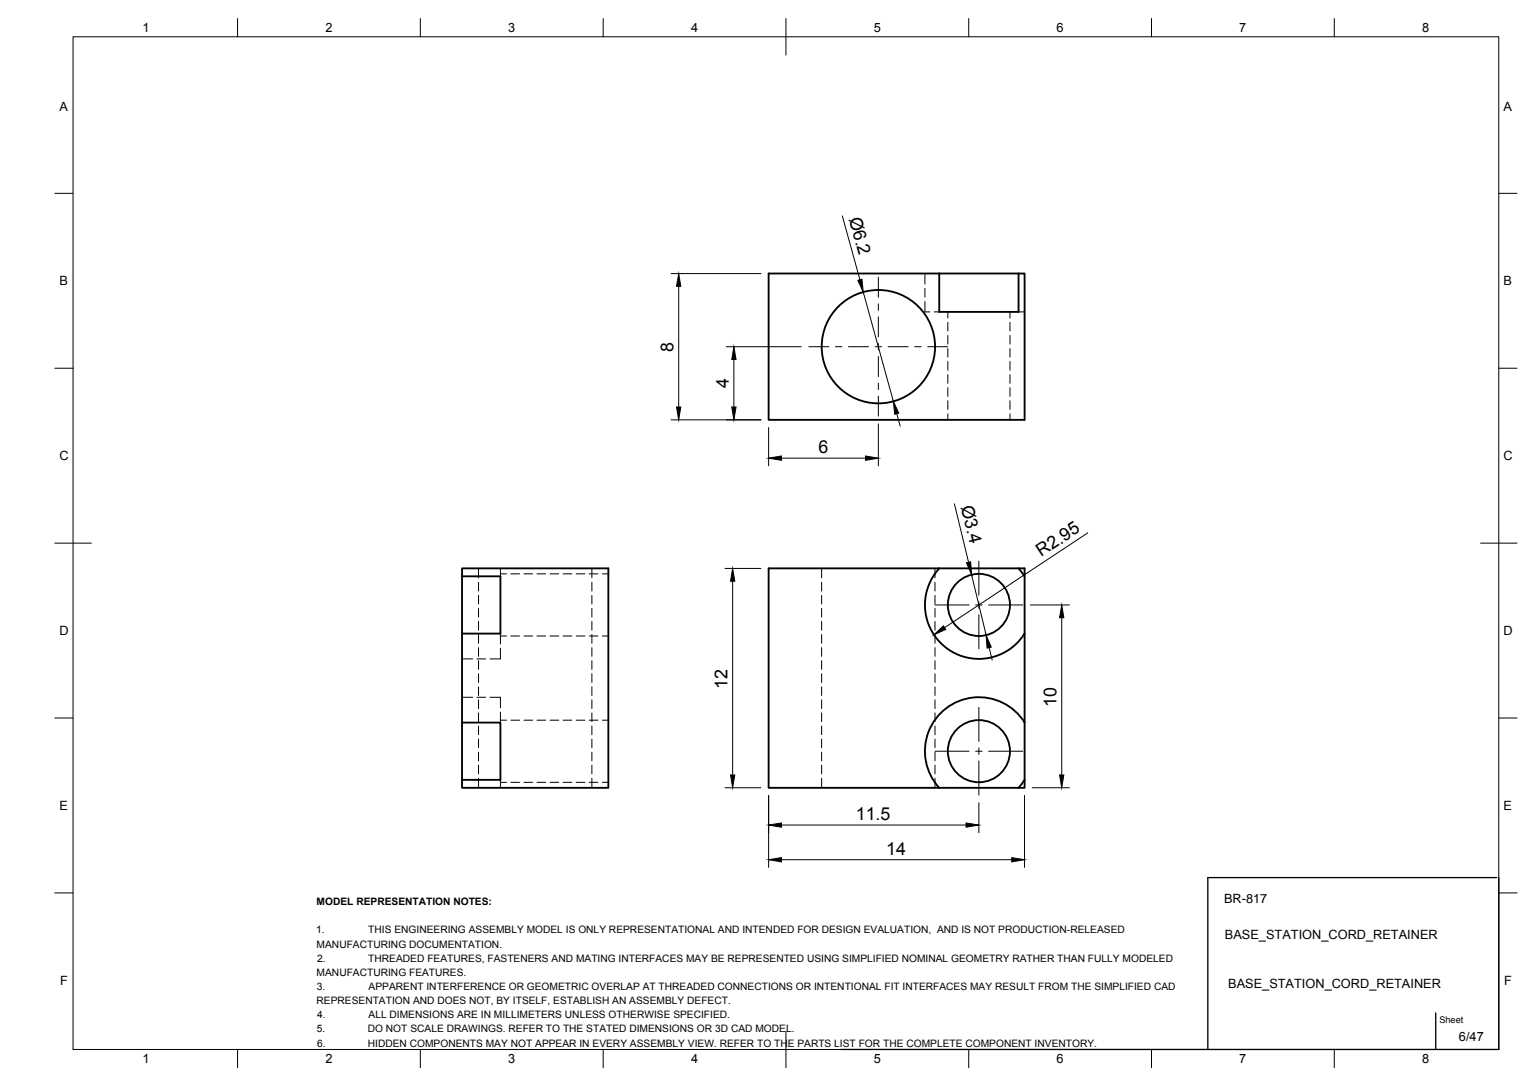
ISO-10303-21;
HEADER;
FILE_DESCRIPTION((''),'2;1');
FILE_NAME('BASE_STATION_CORD_RETAINER.step','2026-10-01T22:07:29-07:00',(''),(''),'','','');
FILE_SCHEMA (('AUTOMOTIVE_DESIGN { 1 0 10303 214 3 1 1 }'));
ENDSEC;
DATA;
#10=MECHANICAL_DESIGN_GEOMETRIC_PRESENTATION_REPRESENTATION('',(#544),#15484);
#474=SHAPE_REPRESENTATION_RELATIONSHIP('SRR','None',#15621,#509) ;
#509=ADVANCED_BREP_SHAPE_REPRESENTATION('',(#586),#15445) ;
#544=STYLED_ITEM('',(#15833),#586) ;
#586=MANIFOLD_SOLID_BREP('BASE_STATION_CORD_RETAINER',#8253) ;
#639=CYLINDRICAL_SURFACE('',#8765,0.295) ;
#640=CYLINDRICAL_SURFACE('',#8771,0.295) ;
#641=CYLINDRICAL_SURFACE('',#8776,0.17) ;
#642=CYLINDRICAL_SURFACE('',#8778,0.295) ;
#643=CYLINDRICAL_SURFACE('',#8781,0.295) ;
#644=CYLINDRICAL_SURFACE('',#8789,0.17) ;
#645=CYLINDRICAL_SURFACE('',#8791,0.31) ;
#831=FACE_BOUND('',#1941,.T.) ;
#832=FACE_BOUND('',#1944,.T.) ;
#833=FACE_BOUND('',#1950,.T.) ;
#834=FACE_BOUND('',#1957,.T.) ;
#835=FACE_BOUND('',#1958,.T.) ;
#836=FACE_BOUND('',#1961,.T.) ;
#911=CIRCLE('',#8766,0.295) ;
#912=CIRCLE('',#8767,0.295) ;
#913=CIRCLE('',#8769,0.295) ;
#914=CIRCLE('',#8770,0.17) ;
#915=CIRCLE('',#8772,0.295) ;
#916=CIRCLE('',#8774,0.31) ;
#917=CIRCLE('',#8777,0.17) ;
#918=CIRCLE('',#8779,0.295) ;
#919=CIRCLE('',#8780,0.295) ;
#920=CIRCLE('',#8782,0.295) ;
#921=CIRCLE('',#8783,0.295) ;
#922=CIRCLE('',#8785,0.17) ;
#923=CIRCLE('',#8790,0.17) ;
#924=CIRCLE('',#8792,0.31) ;
#1418=FACE_OUTER_BOUND('',#1939,.T.) ;
#1419=FACE_OUTER_BOUND('',#1940,.T.) ;
#1420=FACE_OUTER_BOUND('',#1942,.T.) ;
#1421=FACE_OUTER_BOUND('',#1943,.T.) ;
#1422=FACE_OUTER_BOUND('',#1945,.T.) ;
#1423=FACE_OUTER_BOUND('',#1946,.T.) ;
#1424=FACE_OUTER_BOUND('',#1947,.T.) ;
#1425=FACE_OUTER_BOUND('',#1948,.T.) ;
#1426=FACE_OUTER_BOUND('',#1949,.T.) ;
#1427=FACE_OUTER_BOUND('',#1951,.T.) ;
#1428=FACE_OUTER_BOUND('',#1952,.T.) ;
#1429=FACE_OUTER_BOUND('',#1953,.T.) ;
#1430=FACE_OUTER_BOUND('',#1954,.T.) ;
#1431=FACE_OUTER_BOUND('',#1955,.T.) ;
#1432=FACE_OUTER_BOUND('',#1956,.T.) ;
#1433=FACE_OUTER_BOUND('',#1959,.T.) ;
#1434=FACE_OUTER_BOUND('',#1960,.T.) ;
#1939=EDGE_LOOP('',(#5513,#5514,#5515,#5516)) ;
#1940=EDGE_LOOP('',(#5517,#5518,#5519,#5520)) ;
#1941=EDGE_LOOP('',(#5521)) ;
#1942=EDGE_LOOP('',(#5522,#5523,#5524,#5525)) ;
#1943=EDGE_LOOP('',(#5526,#5527,#5528,#5529,#5530,#5531,#5532,#5533)) ;
#1944=EDGE_LOOP('',(#5534)) ;
#1945=EDGE_LOOP('',(#5535,#5536,#5537)) ;
#1946=EDGE_LOOP('',(#5538,#5539,#5540,#5541)) ;
#1947=EDGE_LOOP('',(#5542,#5543,#5544,#5545)) ;
#1948=EDGE_LOOP('',(#5546,#5547,#5548,#5549)) ;
#1949=EDGE_LOOP('',(#5550,#5551,#5552,#5553)) ;
#1950=EDGE_LOOP('',(#5554)) ;
#1951=EDGE_LOOP('',(#5555,#5556,#5557,#5558,#5559,#5560,#5561,#5562,#5563,
#5564,#5565,#5566)) ;
#1952=EDGE_LOOP('',(#5567,#5568,#5569)) ;
#1953=EDGE_LOOP('',(#5570,#5571,#5572,#5573,#5574,#5575)) ;
#1954=EDGE_LOOP('',(#5576,#5577,#5578,#5579)) ;
#1955=EDGE_LOOP('',(#5580,#5581,#5582,#5583)) ;
#1956=EDGE_LOOP('',(#5584,#5585,#5586,#5587)) ;
#1957=EDGE_LOOP('',(#5588)) ;
#1958=EDGE_LOOP('',(#5589)) ;
#1959=EDGE_LOOP('',(#5590,#5591,#5592,#5593)) ;
#1960=EDGE_LOOP('',(#5594,#5595,#5596,#5597,#5598,#5599,#5600,#5601)) ;
#1961=EDGE_LOOP('',(#5602)) ;
#2534=LINE('',#13145,#3008) ;
#2535=LINE('',#13149,#3009) ;
#2536=LINE('',#13153,#3010) ;
#2537=LINE('',#13156,#3011) ;
#2538=LINE('',#13161,#3012) ;
#2539=LINE('',#13164,#3013) ;
#2540=LINE('',#13167,#3014) ;
#2541=LINE('',#13169,#3015) ;
#2542=LINE('',#13171,#3016) ;
#2543=LINE('',#13173,#3017) ;
#2544=LINE('',#13174,#3018) ;
#2545=LINE('',#13178,#3019) ;
#2546=LINE('',#13181,#3020) ;
#2547=LINE('',#13186,#3021) ;
#2548=LINE('',#13190,#3022) ;
#2549=LINE('',#13195,#3023) ;
#2550=LINE('',#13199,#3024) ;
#2551=LINE('',#13202,#3025) ;
#2552=LINE('',#13203,#3026) ;
#2553=LINE('',#13207,#3027) ;
#2554=LINE('',#13209,#3028) ;
#2555=LINE('',#13211,#3029) ;
#2556=LINE('',#13212,#3030) ;
#2557=LINE('',#13214,#3031) ;
#2558=LINE('',#13217,#3032) ;
#2559=LINE('',#13218,#3033) ;
#2560=LINE('',#13221,#3034) ;
#2561=LINE('',#13226,#3035) ;
#2562=LINE('',#13229,#3036) ;
#2563=LINE('',#13230,#3037) ;
#2564=LINE('',#13232,#3038) ;
#3008=VECTOR('',#10187,1.) ;
#3009=VECTOR('',#10190,1.) ;
#3010=VECTOR('',#10195,1.) ;
#3011=VECTOR('',#10198,1.) ;
#3012=VECTOR('',#10203,1.) ;
#3013=VECTOR('',#10206,1.) ;
#3014=VECTOR('',#10209,1.) ;
#3015=VECTOR('',#10210,1.) ;
#3016=VECTOR('',#10211,1.) ;
#3017=VECTOR('',#10212,1.) ;
#3018=VECTOR('',#10213,1.) ;
#3019=VECTOR('',#10218,1.) ;
#3020=VECTOR('',#10221,0.17) ;
#3021=VECTOR('',#10226,1.) ;
#3022=VECTOR('',#10229,1.) ;
#3023=VECTOR('',#10234,1.) ;
#3024=VECTOR('',#10237,1.) ;
#3025=VECTOR('',#10242,1.) ;
#3026=VECTOR('',#10243,1.) ;
#3027=VECTOR('',#10248,1.) ;
#3028=VECTOR('',#10249,1.) ;
#3029=VECTOR('',#10250,1.) ;
#3030=VECTOR('',#10251,1.) ;
#3031=VECTOR('',#10254,1.) ;
#3032=VECTOR('',#10257,1.) ;
#3033=VECTOR('',#10258,1.) ;
#3034=VECTOR('',#10261,0.17) ;
#3035=VECTOR('',#10268,0.31) ;
#3036=VECTOR('',#10271,1.) ;
#3037=VECTOR('',#10272,1.) ;
#3038=VECTOR('',#10275,1.) ;
#3468=VERTEX_POINT('',#13143) ;
#3469=VERTEX_POINT('',#13144) ;
#3470=VERTEX_POINT('',#13146) ;
#3471=VERTEX_POINT('',#13148) ;
#3472=VERTEX_POINT('',#13152) ;
#3473=VERTEX_POINT('',#13154) ;
#3474=VERTEX_POINT('',#13157) ;
#3475=VERTEX_POINT('',#13160) ;
#3476=VERTEX_POINT('',#13162) ;
#3477=VERTEX_POINT('',#13166) ;
#3478=VERTEX_POINT('',#13168) ;
#3479=VERTEX_POINT('',#13170) ;
#3480=VERTEX_POINT('',#13172) ;
#3481=VERTEX_POINT('',#13175) ;
#3482=VERTEX_POINT('',#13180) ;
#3483=VERTEX_POINT('',#13184) ;
#3484=VERTEX_POINT('',#13185) ;
#3485=VERTEX_POINT('',#13187) ;
#3486=VERTEX_POINT('',#13189) ;
#3487=VERTEX_POINT('',#13193) ;
#3488=VERTEX_POINT('',#13194) ;
#3489=VERTEX_POINT('',#13196) ;
#3490=VERTEX_POINT('',#13198) ;
#3491=VERTEX_POINT('',#13204) ;
#3492=VERTEX_POINT('',#13208) ;
#3493=VERTEX_POINT('',#13210) ;
#3494=VERTEX_POINT('',#13216) ;
#3495=VERTEX_POINT('',#13220) ;
#3496=VERTEX_POINT('',#13224) ;
#3497=VERTEX_POINT('',#13228) ;
#4261=EDGE_CURVE('',#3468,#3469,#2534,.T.) ;
#4262=EDGE_CURVE('',#3468,#3470,#911,.T.) ;
#4263=EDGE_CURVE('',#3471,#3470,#2535,.T.) ;
#4264=EDGE_CURVE('',#3469,#3471,#912,.T.) ;
#4265=EDGE_CURVE('',#3472,#3468,#2536,.T.) ;
#4266=EDGE_CURVE('',#3473,#3472,#913,.T.) ;
#4267=EDGE_CURVE('',#3470,#3473,#2537,.T.) ;
#4268=EDGE_CURVE('',#3474,#3474,#914,.T.) ;
#4269=EDGE_CURVE('',#3475,#3472,#2538,.T.) ;
#4270=EDGE_CURVE('',#3476,#3475,#915,.T.) ;
#4271=EDGE_CURVE('',#3473,#3476,#2539,.T.) ;
#4272=EDGE_CURVE('',#3477,#3469,#2540,.T.) ;
#4273=EDGE_CURVE('',#3478,#3477,#2541,.T.) ;
#4274=EDGE_CURVE('',#3479,#3478,#2542,.T.) ;
#4275=EDGE_CURVE('',#3479,#3480,#2543,.T.) ;
#4276=EDGE_CURVE('',#3475,#3480,#2544,.T.) ;
#4277=EDGE_CURVE('',#3481,#3481,#916,.T.) ;
#4278=EDGE_CURVE('',#3471,#3477,#2545,.T.) ;
#4279=EDGE_CURVE('',#3474,#3482,#2546,.T.) ;
#4280=EDGE_CURVE('',#3482,#3482,#917,.T.) ;
#4281=EDGE_CURVE('',#3483,#3484,#2547,.T.) ;
#4282=EDGE_CURVE('',#3485,#3483,#918,.T.) ;
#4283=EDGE_CURVE('',#3486,#3485,#2548,.T.) ;
#4284=EDGE_CURVE('',#3486,#3484,#919,.T.) ;
#4285=EDGE_CURVE('',#3487,#3488,#2549,.T.) ;
#4286=EDGE_CURVE('',#3487,#3489,#920,.T.) ;
#4287=EDGE_CURVE('',#3490,#3489,#2550,.T.) ;
#4288=EDGE_CURVE('',#3488,#3490,#921,.T.) ;
#4289=EDGE_CURVE('',#3484,#3487,#2551,.T.) ;
#4290=EDGE_CURVE('',#3489,#3486,#2552,.T.) ;
#4291=EDGE_CURVE('',#3491,#3491,#922,.T.) ;
#4292=EDGE_CURVE('',#3490,#3476,#2553,.T.) ;
#4293=EDGE_CURVE('',#3492,#3485,#2554,.T.) ;
#4294=EDGE_CURVE('',#3493,#3492,#2555,.T.) ;
#4295=EDGE_CURVE('',#3478,#3493,#2556,.T.) ;
#4296=EDGE_CURVE('',#3483,#3492,#2557,.T.) ;
#4297=EDGE_CURVE('',#3480,#3494,#2558,.T.) ;
#4298=EDGE_CURVE('',#3494,#3488,#2559,.T.) ;
#4299=EDGE_CURVE('',#3491,#3495,#2560,.T.) ;
#4300=EDGE_CURVE('',#3495,#3495,#923,.T.) ;
#4301=EDGE_CURVE('',#3496,#3496,#924,.T.) ;
#4302=EDGE_CURVE('',#3496,#3481,#2561,.T.) ;
#4303=EDGE_CURVE('',#3493,#3497,#2562,.T.) ;
#4304=EDGE_CURVE('',#3497,#3479,#2563,.T.) ;
#4305=EDGE_CURVE('',#3497,#3494,#2564,.T.) ;
#5513=ORIENTED_EDGE('',*,*,#4261,.F.) ;
#5514=ORIENTED_EDGE('',*,*,#4262,.T.) ;
#5515=ORIENTED_EDGE('',*,*,#4263,.F.) ;
#5516=ORIENTED_EDGE('',*,*,#4264,.F.) ;
#5517=ORIENTED_EDGE('',*,*,#4265,.F.) ;
#5518=ORIENTED_EDGE('',*,*,#4266,.F.) ;
#5519=ORIENTED_EDGE('',*,*,#4267,.F.) ;
#5520=ORIENTED_EDGE('',*,*,#4262,.F.) ;
#5521=ORIENTED_EDGE('',*,*,#4268,.F.) ;
#5522=ORIENTED_EDGE('',*,*,#4269,.F.) ;
#5523=ORIENTED_EDGE('',*,*,#4270,.F.) ;
#5524=ORIENTED_EDGE('',*,*,#4271,.F.) ;
#5525=ORIENTED_EDGE('',*,*,#4266,.T.) ;
#5526=ORIENTED_EDGE('',*,*,#4269,.T.) ;
#5527=ORIENTED_EDGE('',*,*,#4265,.T.) ;
#5528=ORIENTED_EDGE('',*,*,#4261,.T.) ;
#5529=ORIENTED_EDGE('',*,*,#4272,.F.) ;
#5530=ORIENTED_EDGE('',*,*,#4273,.F.) ;
#5531=ORIENTED_EDGE('',*,*,#4274,.F.) ;
#5532=ORIENTED_EDGE('',*,*,#4275,.T.) ;
#5533=ORIENTED_EDGE('',*,*,#4276,.F.) ;
#5534=ORIENTED_EDGE('',*,*,#4277,.T.) ;
#5535=ORIENTED_EDGE('',*,*,#4264,.T.) ;
#5536=ORIENTED_EDGE('',*,*,#4278,.T.) ;
#5537=ORIENTED_EDGE('',*,*,#4272,.T.) ;
#5538=ORIENTED_EDGE('',*,*,#4268,.T.) ;
#5539=ORIENTED_EDGE('',*,*,#4279,.T.) ;
#5540=ORIENTED_EDGE('',*,*,#4280,.F.) ;
#5541=ORIENTED_EDGE('',*,*,#4279,.F.) ;
#5542=ORIENTED_EDGE('',*,*,#4281,.F.) ;
#5543=ORIENTED_EDGE('',*,*,#4282,.F.) ;
#5544=ORIENTED_EDGE('',*,*,#4283,.F.) ;
#5545=ORIENTED_EDGE('',*,*,#4284,.T.) ;
#5546=ORIENTED_EDGE('',*,*,#4285,.F.) ;
#5547=ORIENTED_EDGE('',*,*,#4286,.T.) ;
#5548=ORIENTED_EDGE('',*,*,#4287,.F.) ;
#5549=ORIENTED_EDGE('',*,*,#4288,.F.) ;
#5550=ORIENTED_EDGE('',*,*,#4289,.F.) ;
#5551=ORIENTED_EDGE('',*,*,#4284,.F.) ;
#5552=ORIENTED_EDGE('',*,*,#4290,.F.) ;
#5553=ORIENTED_EDGE('',*,*,#4286,.F.) ;
#5554=ORIENTED_EDGE('',*,*,#4291,.F.) ;
#5555=ORIENTED_EDGE('',*,*,#4271,.T.) ;
#5556=ORIENTED_EDGE('',*,*,#4292,.F.) ;
#5557=ORIENTED_EDGE('',*,*,#4287,.T.) ;
#5558=ORIENTED_EDGE('',*,*,#4290,.T.) ;
#5559=ORIENTED_EDGE('',*,*,#4283,.T.) ;
#5560=ORIENTED_EDGE('',*,*,#4293,.F.) ;
#5561=ORIENTED_EDGE('',*,*,#4294,.F.) ;
#5562=ORIENTED_EDGE('',*,*,#4295,.F.) ;
#5563=ORIENTED_EDGE('',*,*,#4273,.T.) ;
#5564=ORIENTED_EDGE('',*,*,#4278,.F.) ;
#5565=ORIENTED_EDGE('',*,*,#4263,.T.) ;
#5566=ORIENTED_EDGE('',*,*,#4267,.T.) ;
#5567=ORIENTED_EDGE('',*,*,#4282,.T.) ;
#5568=ORIENTED_EDGE('',*,*,#4296,.T.) ;
#5569=ORIENTED_EDGE('',*,*,#4293,.T.) ;
#5570=ORIENTED_EDGE('',*,*,#4270,.T.) ;
#5571=ORIENTED_EDGE('',*,*,#4276,.T.) ;
#5572=ORIENTED_EDGE('',*,*,#4297,.T.) ;
#5573=ORIENTED_EDGE('',*,*,#4298,.T.) ;
#5574=ORIENTED_EDGE('',*,*,#4288,.T.) ;
#5575=ORIENTED_EDGE('',*,*,#4292,.T.) ;
#5576=ORIENTED_EDGE('',*,*,#4291,.T.) ;
#5577=ORIENTED_EDGE('',*,*,#4299,.T.) ;
#5578=ORIENTED_EDGE('',*,*,#4300,.F.) ;
#5579=ORIENTED_EDGE('',*,*,#4299,.F.) ;
#5580=ORIENTED_EDGE('',*,*,#4301,.F.) ;
#5581=ORIENTED_EDGE('',*,*,#4302,.T.) ;
#5582=ORIENTED_EDGE('',*,*,#4277,.F.) ;
#5583=ORIENTED_EDGE('',*,*,#4302,.F.) ;
#5584=ORIENTED_EDGE('',*,*,#4274,.T.) ;
#5585=ORIENTED_EDGE('',*,*,#4295,.T.) ;
#5586=ORIENTED_EDGE('',*,*,#4303,.T.) ;
#5587=ORIENTED_EDGE('',*,*,#4304,.T.) ;
#5588=ORIENTED_EDGE('',*,*,#4280,.T.) ;
#5589=ORIENTED_EDGE('',*,*,#4300,.T.) ;
#5590=ORIENTED_EDGE('',*,*,#4305,.T.) ;
#5591=ORIENTED_EDGE('',*,*,#4297,.F.) ;
#5592=ORIENTED_EDGE('',*,*,#4275,.F.) ;
#5593=ORIENTED_EDGE('',*,*,#4304,.F.) ;
#5594=ORIENTED_EDGE('',*,*,#4285,.T.) ;
#5595=ORIENTED_EDGE('',*,*,#4298,.F.) ;
#5596=ORIENTED_EDGE('',*,*,#4305,.F.) ;
#5597=ORIENTED_EDGE('',*,*,#4303,.F.) ;
#5598=ORIENTED_EDGE('',*,*,#4294,.T.) ;
#5599=ORIENTED_EDGE('',*,*,#4296,.F.) ;
#5600=ORIENTED_EDGE('',*,*,#4281,.T.) ;
#5601=ORIENTED_EDGE('',*,*,#4289,.T.) ;
#5602=ORIENTED_EDGE('',*,*,#4301,.T.) ;
#7577=PLANE('',#8768) ;
#7578=PLANE('',#8773) ;
#7579=PLANE('',#8775) ;
#7580=PLANE('',#8784) ;
#7581=PLANE('',#8786) ;
#7582=PLANE('',#8787) ;
#7583=PLANE('',#8788) ;
#7584=PLANE('',#8793) ;
#7585=PLANE('',#8794) ;
#7586=PLANE('',#8795) ;
#7805=ADVANCED_FACE('',(#1418),#639,.F.) ;
#7806=ADVANCED_FACE('',(#1419,#831),#7577,.F.) ;
#7807=ADVANCED_FACE('',(#1420),#640,.F.) ;
#7808=ADVANCED_FACE('',(#1421,#832),#7578,.F.) ;
#7809=ADVANCED_FACE('',(#1422),#7579,.F.) ;
#7810=ADVANCED_FACE('',(#1423),#641,.F.) ;
#7811=ADVANCED_FACE('',(#1424),#642,.F.) ;
#7812=ADVANCED_FACE('',(#1425),#643,.F.) ;
#7813=ADVANCED_FACE('',(#1426,#833),#7580,.F.) ;
#7814=ADVANCED_FACE('',(#1427),#7581,.F.) ;
#7815=ADVANCED_FACE('',(#1428),#7582,.F.) ;
#7816=ADVANCED_FACE('',(#1429),#7583,.F.) ;
#7817=ADVANCED_FACE('',(#1430),#644,.F.) ;
#7818=ADVANCED_FACE('',(#1431),#645,.F.) ;
#7819=ADVANCED_FACE('',(#1432,#834,#835),#7584,.T.) ;
#7820=ADVANCED_FACE('',(#1433),#7585,.F.) ;
#7821=ADVANCED_FACE('',(#1434,#836),#7586,.F.) ;
#8253=CLOSED_SHELL('',(#7805,#7806,#7807,#7808,#7809,#7810,#7811,#7812,
#7813,#7814,#7815,#7816,#7817,#7818,#7819,#7820,#7821)) ;
#8764=AXIS2_PLACEMENT_3D('',#13141,#10183,#10184) ;
#8765=AXIS2_PLACEMENT_3D('',#13142,#10185,#10186) ;
#8766=AXIS2_PLACEMENT_3D('',#13147,#10188,#10189) ;
#8767=AXIS2_PLACEMENT_3D('',#13150,#10191,#10192) ;
#8768=AXIS2_PLACEMENT_3D('',#13151,#10193,#10194) ;
#8769=AXIS2_PLACEMENT_3D('',#13155,#10196,#10197) ;
#8770=AXIS2_PLACEMENT_3D('',#13158,#10199,#10200) ;
#8771=AXIS2_PLACEMENT_3D('',#13159,#10201,#10202) ;
#8772=AXIS2_PLACEMENT_3D('',#13163,#10204,#10205) ;
#8773=AXIS2_PLACEMENT_3D('',#13165,#10207,#10208) ;
#8774=AXIS2_PLACEMENT_3D('',#13176,#10214,#10215) ;
#8775=AXIS2_PLACEMENT_3D('',#13177,#10216,#10217) ;
#8776=AXIS2_PLACEMENT_3D('',#13179,#10219,#10220) ;
#8777=AXIS2_PLACEMENT_3D('',#13182,#10222,#10223) ;
#8778=AXIS2_PLACEMENT_3D('',#13183,#10224,#10225) ;
#8779=AXIS2_PLACEMENT_3D('',#13188,#10227,#10228) ;
#8780=AXIS2_PLACEMENT_3D('',#13191,#10230,#10231) ;
#8781=AXIS2_PLACEMENT_3D('',#13192,#10232,#10233) ;
#8782=AXIS2_PLACEMENT_3D('',#13197,#10235,#10236) ;
#8783=AXIS2_PLACEMENT_3D('',#13200,#10238,#10239) ;
#8784=AXIS2_PLACEMENT_3D('',#13201,#10240,#10241) ;
#8785=AXIS2_PLACEMENT_3D('',#13205,#10244,#10245) ;
#8786=AXIS2_PLACEMENT_3D('',#13206,#10246,#10247) ;
#8787=AXIS2_PLACEMENT_3D('',#13213,#10252,#10253) ;
#8788=AXIS2_PLACEMENT_3D('',#13215,#10255,#10256) ;
#8789=AXIS2_PLACEMENT_3D('',#13219,#10259,#10260) ;
#8790=AXIS2_PLACEMENT_3D('',#13222,#10262,#10263) ;
#8791=AXIS2_PLACEMENT_3D('',#13223,#10264,#10265) ;
#8792=AXIS2_PLACEMENT_3D('',#13225,#10266,#10267) ;
#8793=AXIS2_PLACEMENT_3D('',#13227,#10269,#10270) ;
#8794=AXIS2_PLACEMENT_3D('',#13231,#10273,#10274) ;
#8795=AXIS2_PLACEMENT_3D('',#13233,#10276,#10277) ;
#10183=DIRECTION('axis',(0.,0.,1.)) ;
#10184=DIRECTION('refdir',(1.,0.,0.)) ;
#10185=DIRECTION('center_axis',(0.,0.,1.)) ;
#10186=DIRECTION('ref_axis',(1.,0.,0.)) ;
#10187=DIRECTION('',(0.,0.,-1.)) ;
#10188=DIRECTION('center_axis',(0.,0.,1.)) ;
#10189=DIRECTION('ref_axis',(1.,0.,0.)) ;
#10190=DIRECTION('',(0.,0.,1.)) ;
#10191=DIRECTION('center_axis',(0.,0.,1.)) ;
#10192=DIRECTION('ref_axis',(1.,0.,0.)) ;
#10193=DIRECTION('center_axis',(0.,0.,1.)) ;
#10194=DIRECTION('ref_axis',(1.,0.,0.)) ;
#10195=DIRECTION('',(0.,1.,0.)) ;
#10196=DIRECTION('center_axis',(0.,0.,1.)) ;
#10197=DIRECTION('ref_axis',(1.,0.,0.)) ;
#10198=DIRECTION('',(-1.,0.,0.)) ;
#10199=DIRECTION('center_axis',(0.,0.,-1.)) ;
#10200=DIRECTION('ref_axis',(1.,0.,0.)) ;
#10201=DIRECTION('center_axis',(0.,0.,1.)) ;
#10202=DIRECTION('ref_axis',(-0.794686467668033,-0.60702011342731,0.)) ;
#10203=DIRECTION('',(0.,0.,1.)) ;
#10204=DIRECTION('center_axis',(0.,0.,1.)) ;
#10205=DIRECTION('ref_axis',(1.,0.,0.)) ;
#10206=DIRECTION('',(0.,0.,-1.)) ;
#10207=DIRECTION('center_axis',(-1.,0.,0.)) ;
#10208=DIRECTION('ref_axis',(0.,0.,1.)) ;
#10209=DIRECTION('',(0.,-1.,0.)) ;
#10210=DIRECTION('',(0.,0.,-1.)) ;
#10211=DIRECTION('',(0.,1.,0.)) ;
#10212=DIRECTION('',(0.,0.,-1.)) ;
#10213=DIRECTION('',(0.,-1.,0.)) ;
#10214=DIRECTION('center_axis',(-1.,0.,0.)) ;
#10215=DIRECTION('ref_axis',(0.,0.,-1.)) ;
#10216=DIRECTION('center_axis',(0.,0.,1.)) ;
#10217=DIRECTION('ref_axis',(1.,0.,0.)) ;
#10218=DIRECTION('',(1.,0.,0.)) ;
#10219=DIRECTION('center_axis',(0.,0.,1.)) ;
#10220=DIRECTION('ref_axis',(1.,0.,0.)) ;
#10221=DIRECTION('',(0.,0.,1.)) ;
#10222=DIRECTION('center_axis',(0.,0.,-1.)) ;
#10223=DIRECTION('ref_axis',(1.,0.,0.)) ;
#10224=DIRECTION('center_axis',(0.,0.,1.)) ;
#10225=DIRECTION('ref_axis',(1.,0.,0.)) ;
#10226=DIRECTION('',(0.,0.,1.)) ;
#10227=DIRECTION('center_axis',(0.,0.,1.)) ;
#10228=DIRECTION('ref_axis',(1.,0.,0.)) ;
#10229=DIRECTION('',(0.,0.,-1.)) ;
#10230=DIRECTION('center_axis',(0.,0.,1.)) ;
#10231=DIRECTION('ref_axis',(1.,0.,0.)) ;
#10232=DIRECTION('center_axis',(0.,0.,1.)) ;
#10233=DIRECTION('ref_axis',(1.,0.,0.)) ;
#10234=DIRECTION('',(0.,0.,-1.)) ;
#10235=DIRECTION('center_axis',(0.,0.,1.)) ;
#10236=DIRECTION('ref_axis',(1.,0.,0.)) ;
#10237=DIRECTION('',(0.,0.,1.)) ;
#10238=DIRECTION('center_axis',(0.,0.,1.)) ;
#10239=DIRECTION('ref_axis',(1.,0.,0.)) ;
#10240=DIRECTION('center_axis',(0.,0.,1.)) ;
#10241=DIRECTION('ref_axis',(1.,0.,0.)) ;
#10242=DIRECTION('',(0.,-1.,0.)) ;
#10243=DIRECTION('',(-1.,0.,0.)) ;
#10244=DIRECTION('center_axis',(0.,0.,-1.)) ;
#10245=DIRECTION('ref_axis',(1.,0.,0.)) ;
#10246=DIRECTION('center_axis',(0.,-1.,0.)) ;
#10247=DIRECTION('ref_axis',(0.,0.,-1.)) ;
#10248=DIRECTION('',(1.,0.,0.)) ;
#10249=DIRECTION('',(1.,0.,0.)) ;
#10250=DIRECTION('',(0.,0.,-1.)) ;
#10251=DIRECTION('',(-1.,0.,0.)) ;
#10252=DIRECTION('center_axis',(0.,0.,1.)) ;
#10253=DIRECTION('ref_axis',(1.,0.,0.)) ;
#10254=DIRECTION('',(0.,1.,0.)) ;
#10255=DIRECTION('center_axis',(0.,0.,1.)) ;
#10256=DIRECTION('ref_axis',(1.,0.,0.)) ;
#10257=DIRECTION('',(-1.,0.,0.)) ;
#10258=DIRECTION('',(0.,1.,0.)) ;
#10259=DIRECTION('center_axis',(0.,0.,1.)) ;
#10260=DIRECTION('ref_axis',(1.,0.,0.)) ;
#10261=DIRECTION('',(0.,0.,1.)) ;
#10262=DIRECTION('center_axis',(0.,0.,-1.)) ;
#10263=DIRECTION('ref_axis',(1.,0.,0.)) ;
#10264=DIRECTION('center_axis',(1.,0.,0.)) ;
#10265=DIRECTION('ref_axis',(0.,0.,-1.)) ;
#10266=DIRECTION('center_axis',(1.,0.,0.)) ;
#10267=DIRECTION('ref_axis',(0.,0.,-1.)) ;
#10268=DIRECTION('',(1.,0.,0.)) ;
#10269=DIRECTION('center_axis',(0.,0.,1.)) ;
#10270=DIRECTION('ref_axis',(1.,0.,0.)) ;
#10271=DIRECTION('',(0.,-1.,0.)) ;
#10272=DIRECTION('',(1.,0.,0.)) ;
#10273=DIRECTION('center_axis',(0.,1.,0.)) ;
#10274=DIRECTION('ref_axis',(0.,0.,1.)) ;
#10275=DIRECTION('',(0.,0.,-1.)) ;
#10276=DIRECTION('center_axis',(1.,0.,0.)) ;
#10277=DIRECTION('ref_axis',(0.,0.,-1.)) ;
#13141=CARTESIAN_POINT('',(0.,0.,0.)) ;
#13142=CARTESIAN_POINT('Origin',(3.6,-1.05,-0.745)) ;
#13143=CARTESIAN_POINT('',(3.8,-0.833147515577986,-0.59)) ;
#13144=CARTESIAN_POINT('',(3.8,-0.833147515577986,-0.8)) ;
#13145=CARTESIAN_POINT('',(3.8,-0.833147515577986,-0.745)) ;
#13146=CARTESIAN_POINT('',(3.75660459763366,-0.8,-0.59)) ;
#13147=CARTESIAN_POINT('Origin',(3.6,-1.05,-0.59)) ;
#13148=CARTESIAN_POINT('',(3.75660459763366,-0.8,-0.8)) ;
#13149=CARTESIAN_POINT('',(3.75660459763366,-0.8,-0.745)) ;
#13150=CARTESIAN_POINT('Origin',(3.6,-1.05,-0.8)) ;
#13151=CARTESIAN_POINT('Origin',(3.6,-1.05,-0.59)) ;
#13152=CARTESIAN_POINT('',(3.8,-1.26685248442201,-0.59)) ;
#13153=CARTESIAN_POINT('',(3.8,-1.275,-0.59)) ;
#13154=CARTESIAN_POINT('',(3.44339540236634,-0.8,-0.59)) ;
#13155=CARTESIAN_POINT('Origin',(3.6,-1.05,-0.59)) ;
#13156=CARTESIAN_POINT('',(3.4,-0.8,-0.59)) ;
#13157=CARTESIAN_POINT('',(3.43,-1.05,-0.59)) ;
#13158=CARTESIAN_POINT('Origin',(3.6,-1.05,-0.59)) ;
#13159=CARTESIAN_POINT('Origin',(3.6,-1.05,-0.745)) ;
#13160=CARTESIAN_POINT('',(3.8,-1.26685248442201,-0.8)) ;
#13161=CARTESIAN_POINT('',(3.8,-1.26685248442201,-0.745)) ;
#13162=CARTESIAN_POINT('',(3.44339540236634,-0.8,-0.8)) ;
#13163=CARTESIAN_POINT('Origin',(3.6,-1.05,-0.8)) ;
#13164=CARTESIAN_POINT('',(3.44339540236634,-0.8,-0.745)) ;
#13165=CARTESIAN_POINT('Origin',(3.8,-1.5,-0.4)) ;
#13166=CARTESIAN_POINT('',(3.8,-0.8,-0.8)) ;
#13167=CARTESIAN_POINT('',(3.8,-1.5,-0.8)) ;
#13168=CARTESIAN_POINT('',(3.8,-0.8,0.)) ;
#13169=CARTESIAN_POINT('',(3.8,-0.8,-0.4)) ;
#13170=CARTESIAN_POINT('',(3.8,-2.2,0.)) ;
#13171=CARTESIAN_POINT('',(3.8,-1.5,0.)) ;
#13172=CARTESIAN_POINT('',(3.8,-2.2,-0.8)) ;
#13173=CARTESIAN_POINT('',(3.8,-2.2,-0.4)) ;
#13174=CARTESIAN_POINT('',(3.8,-1.5,-0.8)) ;
#13175=CARTESIAN_POINT('',(3.8,-1.6,-0.09)) ;
#13176=CARTESIAN_POINT('Origin',(3.8,-1.6,-0.4)) ;
#13177=CARTESIAN_POINT('Origin',(3.2,-1.5,-0.8)) ;
#13178=CARTESIAN_POINT('',(3.2,-0.8,-0.8)) ;
#13179=CARTESIAN_POINT('Origin',(3.6,-1.05,-0.4)) ;
#13180=CARTESIAN_POINT('',(3.43,-1.05,0.)) ;
#13181=CARTESIAN_POINT('',(3.43,-1.05,-0.4)) ;
#13182=CARTESIAN_POINT('Origin',(3.6,-1.05,0.)) ;
#13183=CARTESIAN_POINT('Origin',(2.8,-1.05,-0.745)) ;
#13184=CARTESIAN_POINT('',(2.6,-0.833147515577986,-0.8)) ;
#13185=CARTESIAN_POINT('',(2.6,-0.833147515577986,-0.59)) ;
#13186=CARTESIAN_POINT('',(2.6,-0.833147515577986,-0.745)) ;
#13187=CARTESIAN_POINT('',(2.64339540236634,-0.8,-0.8)) ;
#13188=CARTESIAN_POINT('Origin',(2.8,-1.05,-0.8)) ;
#13189=CARTESIAN_POINT('',(2.64339540236634,-0.8,-0.59)) ;
#13190=CARTESIAN_POINT('',(2.64339540236634,-0.8,-0.745)) ;
#13191=CARTESIAN_POINT('Origin',(2.8,-1.05,-0.59)) ;
#13192=CARTESIAN_POINT('Origin',(2.8,-1.05,-0.745)) ;
#13193=CARTESIAN_POINT('',(2.6,-1.26685248442201,-0.59)) ;
#13194=CARTESIAN_POINT('',(2.6,-1.26685248442201,-0.8)) ;
#13195=CARTESIAN_POINT('',(2.6,-1.26685248442201,-0.745)) ;
#13196=CARTESIAN_POINT('',(2.95660459763366,-0.8,-0.59)) ;
#13197=CARTESIAN_POINT('Origin',(2.8,-1.05,-0.59)) ;
#13198=CARTESIAN_POINT('',(2.95660459763366,-0.8,-0.8)) ;
#13199=CARTESIAN_POINT('',(2.95660459763366,-0.8,-0.745)) ;
#13200=CARTESIAN_POINT('Origin',(2.8,-1.05,-0.8)) ;
#13201=CARTESIAN_POINT('Origin',(2.8,-1.05,-0.59)) ;
#13202=CARTESIAN_POINT('',(2.6,-1.275,-0.59)) ;
#13203=CARTESIAN_POINT('',(3.,-0.8,-0.59)) ;
#13204=CARTESIAN_POINT('',(2.63,-1.05,-0.59)) ;
#13205=CARTESIAN_POINT('Origin',(2.8,-1.05,-0.59)) ;
#13206=CARTESIAN_POINT('Origin',(3.2,-0.8,-0.4)) ;
#13207=CARTESIAN_POINT('',(3.2,-0.8,-0.8)) ;
#13208=CARTESIAN_POINT('',(2.6,-0.8,-0.8)) ;
#13209=CARTESIAN_POINT('',(3.2,-0.8,-0.8)) ;
#13210=CARTESIAN_POINT('',(2.6,-0.8,0.)) ;
#13211=CARTESIAN_POINT('',(2.6,-0.8,-0.4)) ;
#13212=CARTESIAN_POINT('',(3.2,-0.8,0.)) ;
#13213=CARTESIAN_POINT('Origin',(3.2,-1.5,-0.8)) ;
#13214=CARTESIAN_POINT('',(2.6,-1.5,-0.8)) ;
#13215=CARTESIAN_POINT('Origin',(3.2,-1.5,-0.8)) ;
#13216=CARTESIAN_POINT('',(2.6,-2.2,-0.8)) ;
#13217=CARTESIAN_POINT('',(3.2,-2.2,-0.8)) ;
#13218=CARTESIAN_POINT('',(2.6,-1.5,-0.8)) ;
#13219=CARTESIAN_POINT('Origin',(2.8,-1.05,-0.4)) ;
#13220=CARTESIAN_POINT('',(2.63,-1.05,0.)) ;
#13221=CARTESIAN_POINT('',(2.63,-1.05,-0.4)) ;
#13222=CARTESIAN_POINT('Origin',(2.8,-1.05,0.)) ;
#13223=CARTESIAN_POINT('Origin',(3.2,-1.6,-0.4)) ;
#13224=CARTESIAN_POINT('',(2.6,-1.6,-0.09)) ;
#13225=CARTESIAN_POINT('Origin',(2.6,-1.6,-0.4)) ;
#13226=CARTESIAN_POINT('',(3.2,-1.6,-0.09)) ;
#13227=CARTESIAN_POINT('Origin',(3.2,-1.5,0.)) ;
#13228=CARTESIAN_POINT('',(2.6,-2.2,0.)) ;
#13229=CARTESIAN_POINT('',(2.6,-1.5,0.)) ;
#13230=CARTESIAN_POINT('',(3.2,-2.2,0.)) ;
#13231=CARTESIAN_POINT('Origin',(3.2,-2.2,-0.4)) ;
#13232=CARTESIAN_POINT('',(2.6,-2.2,-0.4)) ;
#13233=CARTESIAN_POINT('Origin',(2.6,-1.5,-0.4)) ;
#15402=UNCERTAINTY_MEASURE_WITH_UNIT(LENGTH_MEASURE(0.001),#15485,
'DISTANCE_ACCURACY_VALUE',
'Maximum model space distance between geometric entities at asserted c
onnectivities') ;
#15441=UNCERTAINTY_MEASURE_WITH_UNIT(LENGTH_MEASURE(0.001),#15485,
'DISTANCE_ACCURACY_VALUE',
'Maximum model space distance between geometric entities at asserted c
onnectivities') ;
#15445=(
GEOMETRIC_REPRESENTATION_CONTEXT(3)
GLOBAL_UNCERTAINTY_ASSIGNED_CONTEXT((#15402))
GLOBAL_UNIT_ASSIGNED_CONTEXT((#15485,#15487,#15488))
REPRESENTATION_CONTEXT('','3D')
) ;
#15484=(
GEOMETRIC_REPRESENTATION_CONTEXT(3)
GLOBAL_UNCERTAINTY_ASSIGNED_CONTEXT((#15441))
GLOBAL_UNIT_ASSIGNED_CONTEXT((#15485,#15487,#15488))
REPRESENTATION_CONTEXT('','3D')
) ;
#15485=(
LENGTH_UNIT()
NAMED_UNIT(*)
SI_UNIT(.CENTI.,.METRE.)
) ;
#15487=(
NAMED_UNIT(*)
PLANE_ANGLE_UNIT()
SI_UNIT($,.RADIAN.)
) ;
#15488=(
NAMED_UNIT(*)
SI_UNIT($,.STERADIAN.)
SOLID_ANGLE_UNIT()
) ;
#15492=SHAPE_DEFINITION_REPRESENTATION(#15534,#15621) ;
#15534=PRODUCT_DEFINITION_SHAPE('',$,#15664) ;
#15621=SHAPE_REPRESENTATION('',(#8764),#15445) ;
#15660=PRODUCT_DEFINITION_CONTEXT('part definition',#15788,'design') ;
#15664=PRODUCT_DEFINITION('BASE_STATION_CORD_RETAINER',
'BASE_STATION_CORD_RETAINER',#15706,#15660) ;
#15706=PRODUCT_DEFINITION_FORMATION('',$,#15793) ;
#15788=APPLICATION_CONTEXT(
'Core Data for Automotive Mechanical Design Process') ;
#15789=PRODUCT_CONTEXT('part definition',#15788,'mechanical') ;
#15793=PRODUCT('BASE_STATION_CORD_RETAINER','BASE_STATION_CORD_RETAINER',$,
(#15789)) ;
#15833=PRESENTATION_STYLE_ASSIGNMENT((#15845)) ;
#15845=SURFACE_STYLE_USAGE(.BOTH.,#15857) ;
#15857=SURFACE_SIDE_STYLE('',(#15869)) ;
#15869=SURFACE_STYLE_FILL_AREA(#15881) ;
#15881=FILL_AREA_STYLE('Nylon 6-6 (White)',(#15893)) ;
#15893=FILL_AREA_STYLE_COLOUR('Nylon 6-6 (White)',#15905) ;
#15905=COLOUR_RGB('Nylon 6-6 (White)', 0.31764706, 0.68627451, 0.89019608) ;
ENDSEC;
END-ISO-10303-21;
